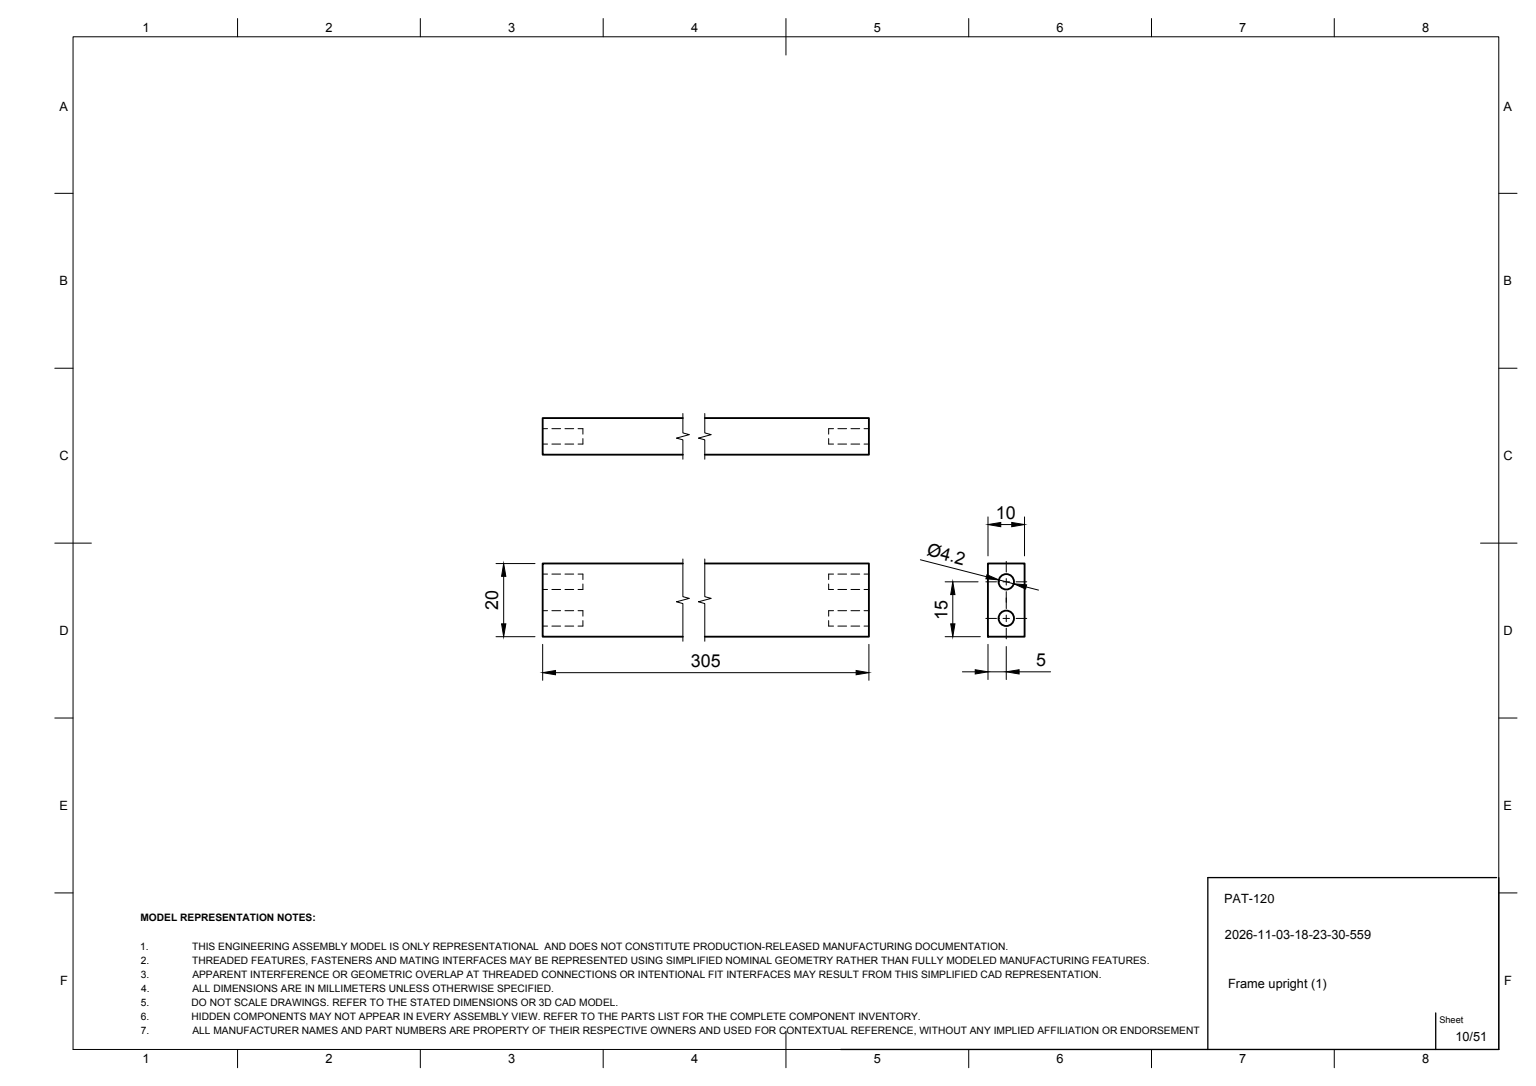
ISO-10303-21;
HEADER;
/* Generated by software containing ST-Developer
 * from STEP Tools, Inc. (www.steptools.com) 
 */

FILE_DESCRIPTION(
/* description */ ('Vibration shaker table dummy'),
/* implementation_level */ '2;1');

FILE_NAME(
/* name */ 'Frame upright (1).step',
/* time_stamp */ '2026-10-27T10:55:14-07:00',
/* author */ (''),
/* organization */ (''),
/* preprocessor_version */ 'ST-DEVELOPER v20.2',
/* originating_system */ 'Autodesk Translation Framework v15.17.0.0',
/* authorisation */ '');

FILE_SCHEMA (('AUTOMOTIVE_DESIGN { 1 0 10303 214 3 1 1 }'));
ENDSEC;

DATA;
#10=MECHANICAL_DESIGN_GEOMETRIC_PRESENTATION_REPRESENTATION('',(#691),#22394);
#599=SHAPE_REPRESENTATION_RELATIONSHIP('SRR','None',#22645,#645);
#645=ADVANCED_BREP_SHAPE_REPRESENTATION('',(#737),#22351);
#691=STYLED_ITEM('',(#22940),#737);
#737=MANIFOLD_SOLID_BREP('Body1',#9209);
#859=FACE_BOUND('',#2014,.T.);
#860=FACE_BOUND('',#2015,.T.);
#861=FACE_BOUND('',#2017,.T.);
#862=FACE_BOUND('',#2018,.T.);
#1094=PLANE('',#9937);
#1095=PLANE('',#9941);
#1096=PLANE('',#9945);
#1097=PLANE('',#9949);
#1098=PLANE('',#9950);
#1099=PLANE('',#9951);
#1100=PLANE('',#9952);
#1101=PLANE('',#9953);
#1102=PLANE('',#9954);
#1103=PLANE('',#9955);
#1419=FACE_OUTER_BOUND('',#2001,.T.);
#1420=FACE_OUTER_BOUND('',#2002,.T.);
#1421=FACE_OUTER_BOUND('',#2003,.T.);
#1422=FACE_OUTER_BOUND('',#2004,.T.);
#1423=FACE_OUTER_BOUND('',#2005,.T.);
#1424=FACE_OUTER_BOUND('',#2006,.T.);
#1425=FACE_OUTER_BOUND('',#2007,.T.);
#1426=FACE_OUTER_BOUND('',#2008,.T.);
#1427=FACE_OUTER_BOUND('',#2009,.T.);
#1428=FACE_OUTER_BOUND('',#2010,.T.);
#1429=FACE_OUTER_BOUND('',#2011,.T.);
#1430=FACE_OUTER_BOUND('',#2012,.T.);
#1431=FACE_OUTER_BOUND('',#2013,.T.);
#1432=FACE_OUTER_BOUND('',#2016,.T.);
#2001=EDGE_LOOP('',(#6630,#6631,#6632,#6633));
#2002=EDGE_LOOP('',(#6634));
#2003=EDGE_LOOP('',(#6635,#6636,#6637,#6638));
#2004=EDGE_LOOP('',(#6639));
#2005=EDGE_LOOP('',(#6640,#6641,#6642,#6643));
#2006=EDGE_LOOP('',(#6644));
#2007=EDGE_LOOP('',(#6645,#6646,#6647,#6648));
#2008=EDGE_LOOP('',(#6649));
#2009=EDGE_LOOP('',(#6650,#6651,#6652,#6653));
#2010=EDGE_LOOP('',(#6654,#6655,#6656,#6657));
#2011=EDGE_LOOP('',(#6658,#6659,#6660,#6661));
#2012=EDGE_LOOP('',(#6662,#6663,#6664,#6665));
#2013=EDGE_LOOP('',(#6666,#6667,#6668,#6669));
#2014=EDGE_LOOP('',(#6670));
#2015=EDGE_LOOP('',(#6671));
#2016=EDGE_LOOP('',(#6672,#6673,#6674,#6675));
#2017=EDGE_LOOP('',(#6676));
#2018=EDGE_LOOP('',(#6677));
#2726=LINE('',#14359,#3345);
#2727=LINE('',#14366,#3346);
#2728=LINE('',#14373,#3347);
#2729=LINE('',#14380,#3348);
#2730=LINE('',#14386,#3349);
#2731=LINE('',#14388,#3350);
#2732=LINE('',#14390,#3351);
#2733=LINE('',#14391,#3352);
#2734=LINE('',#14394,#3353);
#2735=LINE('',#14396,#3354);
#2736=LINE('',#14397,#3355);
#2737=LINE('',#14400,#3356);
#2738=LINE('',#14402,#3357);
#2739=LINE('',#14403,#3358);
#2740=LINE('',#14405,#3359);
#2741=LINE('',#14406,#3360);
#3345=VECTOR('',#11406,0.210000000000001);
#3346=VECTOR('',#11415,0.210000000000001);
#3347=VECTOR('',#11424,0.210000000000001);
#3348=VECTOR('',#11433,0.210000000000001);
#3349=VECTOR('',#11440,1.);
#3350=VECTOR('',#11441,1.);
#3351=VECTOR('',#11442,1.);
#3352=VECTOR('',#11443,1.);
#3353=VECTOR('',#11446,1.);
#3354=VECTOR('',#11447,1.);
#3355=VECTOR('',#11448,1.);
#3356=VECTOR('',#11451,1.);
#3357=VECTOR('',#11452,1.);
#3358=VECTOR('',#11453,1.);
#3359=VECTOR('',#11456,1.);
#3360=VECTOR('',#11457,1.);
#3948=CIRCLE('',#9935,0.210000000000001);
#3949=CIRCLE('',#9936,0.210000000000001);
#3950=CIRCLE('',#9939,0.210000000000001);
#3951=CIRCLE('',#9940,0.210000000000001);
#3952=CIRCLE('',#9943,0.210000000000001);
#3953=CIRCLE('',#9944,0.210000000000001);
#3954=CIRCLE('',#9947,0.210000000000001);
#3955=CIRCLE('',#9948,0.210000000000001);
#4495=VERTEX_POINT('',#14356);
#4496=VERTEX_POINT('',#14358);
#4497=VERTEX_POINT('',#14363);
#4498=VERTEX_POINT('',#14365);
#4499=VERTEX_POINT('',#14370);
#4500=VERTEX_POINT('',#14372);
#4501=VERTEX_POINT('',#14377);
#4502=VERTEX_POINT('',#14379);
#4503=VERTEX_POINT('',#14384);
#4504=VERTEX_POINT('',#14385);
#4505=VERTEX_POINT('',#14387);
#4506=VERTEX_POINT('',#14389);
#4507=VERTEX_POINT('',#14393);
#4508=VERTEX_POINT('',#14395);
#4509=VERTEX_POINT('',#14399);
#4510=VERTEX_POINT('',#14401);
#5308=EDGE_CURVE('',#4495,#4495,#3948,.T.);
#5309=EDGE_CURVE('',#4495,#4496,#2726,.T.);
#5310=EDGE_CURVE('',#4496,#4496,#3949,.T.);
#5311=EDGE_CURVE('',#4497,#4497,#3950,.T.);
#5312=EDGE_CURVE('',#4497,#4498,#2727,.T.);
#5313=EDGE_CURVE('',#4498,#4498,#3951,.T.);
#5314=EDGE_CURVE('',#4499,#4499,#3952,.T.);
#5315=EDGE_CURVE('',#4499,#4500,#2728,.T.);
#5316=EDGE_CURVE('',#4500,#4500,#3953,.T.);
#5317=EDGE_CURVE('',#4501,#4501,#3954,.T.);
#5318=EDGE_CURVE('',#4501,#4502,#2729,.T.);
#5319=EDGE_CURVE('',#4502,#4502,#3955,.T.);
#5320=EDGE_CURVE('',#4503,#4504,#2730,.T.);
#5321=EDGE_CURVE('',#4504,#4505,#2731,.T.);
#5322=EDGE_CURVE('',#4506,#4505,#2732,.T.);
#5323=EDGE_CURVE('',#4503,#4506,#2733,.T.);
#5324=EDGE_CURVE('',#4507,#4503,#2734,.T.);
#5325=EDGE_CURVE('',#4508,#4506,#2735,.T.);
#5326=EDGE_CURVE('',#4507,#4508,#2736,.T.);
#5327=EDGE_CURVE('',#4509,#4507,#2737,.T.);
#5328=EDGE_CURVE('',#4510,#4508,#2738,.T.);
#5329=EDGE_CURVE('',#4509,#4510,#2739,.T.);
#5330=EDGE_CURVE('',#4504,#4509,#2740,.T.);
#5331=EDGE_CURVE('',#4505,#4510,#2741,.T.);
#6630=ORIENTED_EDGE('',*,*,#5308,.F.);
#6631=ORIENTED_EDGE('',*,*,#5309,.T.);
#6632=ORIENTED_EDGE('',*,*,#5310,.F.);
#6633=ORIENTED_EDGE('',*,*,#5309,.F.);
#6634=ORIENTED_EDGE('',*,*,#5308,.T.);
#6635=ORIENTED_EDGE('',*,*,#5311,.F.);
#6636=ORIENTED_EDGE('',*,*,#5312,.T.);
#6637=ORIENTED_EDGE('',*,*,#5313,.F.);
#6638=ORIENTED_EDGE('',*,*,#5312,.F.);
#6639=ORIENTED_EDGE('',*,*,#5311,.T.);
#6640=ORIENTED_EDGE('',*,*,#5314,.F.);
#6641=ORIENTED_EDGE('',*,*,#5315,.T.);
#6642=ORIENTED_EDGE('',*,*,#5316,.T.);
#6643=ORIENTED_EDGE('',*,*,#5315,.F.);
#6644=ORIENTED_EDGE('',*,*,#5316,.F.);
#6645=ORIENTED_EDGE('',*,*,#5317,.F.);
#6646=ORIENTED_EDGE('',*,*,#5318,.T.);
#6647=ORIENTED_EDGE('',*,*,#5319,.T.);
#6648=ORIENTED_EDGE('',*,*,#5318,.F.);
#6649=ORIENTED_EDGE('',*,*,#5319,.F.);
#6650=ORIENTED_EDGE('',*,*,#5320,.T.);
#6651=ORIENTED_EDGE('',*,*,#5321,.T.);
#6652=ORIENTED_EDGE('',*,*,#5322,.F.);
#6653=ORIENTED_EDGE('',*,*,#5323,.F.);
#6654=ORIENTED_EDGE('',*,*,#5324,.T.);
#6655=ORIENTED_EDGE('',*,*,#5323,.T.);
#6656=ORIENTED_EDGE('',*,*,#5325,.F.);
#6657=ORIENTED_EDGE('',*,*,#5326,.F.);
#6658=ORIENTED_EDGE('',*,*,#5327,.T.);
#6659=ORIENTED_EDGE('',*,*,#5326,.T.);
#6660=ORIENTED_EDGE('',*,*,#5328,.F.);
#6661=ORIENTED_EDGE('',*,*,#5329,.F.);
#6662=ORIENTED_EDGE('',*,*,#5330,.T.);
#6663=ORIENTED_EDGE('',*,*,#5329,.T.);
#6664=ORIENTED_EDGE('',*,*,#5331,.F.);
#6665=ORIENTED_EDGE('',*,*,#5321,.F.);
#6666=ORIENTED_EDGE('',*,*,#5331,.T.);
#6667=ORIENTED_EDGE('',*,*,#5328,.T.);
#6668=ORIENTED_EDGE('',*,*,#5325,.T.);
#6669=ORIENTED_EDGE('',*,*,#5322,.T.);
#6670=ORIENTED_EDGE('',*,*,#5310,.T.);
#6671=ORIENTED_EDGE('',*,*,#5313,.T.);
#6672=ORIENTED_EDGE('',*,*,#5330,.F.);
#6673=ORIENTED_EDGE('',*,*,#5320,.F.);
#6674=ORIENTED_EDGE('',*,*,#5324,.F.);
#6675=ORIENTED_EDGE('',*,*,#5327,.F.);
#6676=ORIENTED_EDGE('',*,*,#5314,.T.);
#6677=ORIENTED_EDGE('',*,*,#5317,.T.);
#8550=CYLINDRICAL_SURFACE('',#9934,0.210000000000001);
#8551=CYLINDRICAL_SURFACE('',#9938,0.210000000000001);
#8552=CYLINDRICAL_SURFACE('',#9942,0.210000000000001);
#8553=CYLINDRICAL_SURFACE('',#9946,0.210000000000001);
#8784=ADVANCED_FACE('',(#1419),#8550,.F.);
#8785=ADVANCED_FACE('',(#1420),#1094,.T.);
#8786=ADVANCED_FACE('',(#1421),#8551,.F.);
#8787=ADVANCED_FACE('',(#1422),#1095,.T.);
#8788=ADVANCED_FACE('',(#1423),#8552,.F.);
#8789=ADVANCED_FACE('',(#1424),#1096,.F.);
#8790=ADVANCED_FACE('',(#1425),#8553,.F.);
#8791=ADVANCED_FACE('',(#1426),#1097,.F.);
#8792=ADVANCED_FACE('',(#1427),#1098,.T.);
#8793=ADVANCED_FACE('',(#1428),#1099,.T.);
#8794=ADVANCED_FACE('',(#1429),#1100,.T.);
#8795=ADVANCED_FACE('',(#1430),#1101,.T.);
#8796=ADVANCED_FACE('',(#1431,#859,#860),#1102,.T.);
#8797=ADVANCED_FACE('',(#1432,#861,#862),#1103,.F.);
#9209=CLOSED_SHELL('',(#8784,#8785,#8786,#8787,#8788,#8789,#8790,#8791,
#8792,#8793,#8794,#8795,#8796,#8797));
#9933=AXIS2_PLACEMENT_3D('',#14354,#11400,#11401);
#9934=AXIS2_PLACEMENT_3D('',#14355,#11402,#11403);
#9935=AXIS2_PLACEMENT_3D('',#14357,#11404,#11405);
#9936=AXIS2_PLACEMENT_3D('',#14360,#11407,#11408);
#9937=AXIS2_PLACEMENT_3D('',#14361,#11409,#11410);
#9938=AXIS2_PLACEMENT_3D('',#14362,#11411,#11412);
#9939=AXIS2_PLACEMENT_3D('',#14364,#11413,#11414);
#9940=AXIS2_PLACEMENT_3D('',#14367,#11416,#11417);
#9941=AXIS2_PLACEMENT_3D('',#14368,#11418,#11419);
#9942=AXIS2_PLACEMENT_3D('',#14369,#11420,#11421);
#9943=AXIS2_PLACEMENT_3D('',#14371,#11422,#11423);
#9944=AXIS2_PLACEMENT_3D('',#14374,#11425,#11426);
#9945=AXIS2_PLACEMENT_3D('',#14375,#11427,#11428);
#9946=AXIS2_PLACEMENT_3D('',#14376,#11429,#11430);
#9947=AXIS2_PLACEMENT_3D('',#14378,#11431,#11432);
#9948=AXIS2_PLACEMENT_3D('',#14381,#11434,#11435);
#9949=AXIS2_PLACEMENT_3D('',#14382,#11436,#11437);
#9950=AXIS2_PLACEMENT_3D('',#14383,#11438,#11439);
#9951=AXIS2_PLACEMENT_3D('',#14392,#11444,#11445);
#9952=AXIS2_PLACEMENT_3D('',#14398,#11449,#11450);
#9953=AXIS2_PLACEMENT_3D('',#14404,#11454,#11455);
#9954=AXIS2_PLACEMENT_3D('',#14407,#11458,#11459);
#9955=AXIS2_PLACEMENT_3D('',#14408,#11460,#11461);
#11400=DIRECTION('axis',(0.,0.,1.));
#11401=DIRECTION('refdir',(1.,0.,0.));
#11402=DIRECTION('center_axis',(0.,0.,1.));
#11403=DIRECTION('ref_axis',(1.,0.,0.));
#11404=DIRECTION('center_axis',(0.,0.,1.));
#11405=DIRECTION('ref_axis',(1.,0.,0.));
#11406=DIRECTION('',(0.,0.,1.));
#11407=DIRECTION('center_axis',(0.,0.,-1.));
#11408=DIRECTION('ref_axis',(1.,0.,0.));
#11409=DIRECTION('center_axis',(0.,0.,1.));
#11410=DIRECTION('ref_axis',(1.,0.,0.));
#11411=DIRECTION('center_axis',(0.,0.,1.));
#11412=DIRECTION('ref_axis',(1.,0.,0.));
#11413=DIRECTION('center_axis',(0.,0.,1.));
#11414=DIRECTION('ref_axis',(1.,0.,0.));
#11415=DIRECTION('',(0.,0.,1.));
#11416=DIRECTION('center_axis',(0.,0.,-1.));
#11417=DIRECTION('ref_axis',(1.,0.,0.));
#11418=DIRECTION('center_axis',(0.,0.,1.));
#11419=DIRECTION('ref_axis',(1.,0.,0.));
#11420=DIRECTION('center_axis',(0.,0.,1.));
#11421=DIRECTION('ref_axis',(1.,0.,0.));
#11422=DIRECTION('center_axis',(0.,0.,1.));
#11423=DIRECTION('ref_axis',(1.,0.,0.));
#11424=DIRECTION('',(0.,0.,1.));
#11425=DIRECTION('center_axis',(0.,0.,1.));
#11426=DIRECTION('ref_axis',(1.,0.,0.));
#11427=DIRECTION('center_axis',(0.,0.,1.));
#11428=DIRECTION('ref_axis',(1.,0.,0.));
#11429=DIRECTION('center_axis',(0.,0.,1.));
#11430=DIRECTION('ref_axis',(1.,0.,0.));
#11431=DIRECTION('center_axis',(0.,0.,1.));
#11432=DIRECTION('ref_axis',(1.,0.,0.));
#11433=DIRECTION('',(0.,0.,1.));
#11434=DIRECTION('center_axis',(0.,0.,1.));
#11435=DIRECTION('ref_axis',(1.,0.,0.));
#11436=DIRECTION('center_axis',(0.,0.,1.));
#11437=DIRECTION('ref_axis',(1.,0.,0.));
#11438=DIRECTION('center_axis',(0.,1.,0.));
#11439=DIRECTION('ref_axis',(-1.,0.,0.));
#11440=DIRECTION('',(-1.,0.,0.));
#11441=DIRECTION('',(0.,0.,1.));
#11442=DIRECTION('',(-1.,0.,0.));
#11443=DIRECTION('',(0.,0.,1.));
#11444=DIRECTION('center_axis',(1.,0.,0.));
#11445=DIRECTION('ref_axis',(0.,1.,0.));
#11446=DIRECTION('',(0.,1.,0.));
#11447=DIRECTION('',(0.,1.,0.));
#11448=DIRECTION('',(0.,0.,1.));
#11449=DIRECTION('center_axis',(0.,-1.,0.));
#11450=DIRECTION('ref_axis',(1.,0.,0.));
#11451=DIRECTION('',(1.,0.,0.));
#11452=DIRECTION('',(1.,0.,0.));
#11453=DIRECTION('',(0.,0.,1.));
#11454=DIRECTION('center_axis',(-1.,0.,0.));
#11455=DIRECTION('ref_axis',(0.,-1.,0.));
#11456=DIRECTION('',(0.,-1.,0.));
#11457=DIRECTION('',(0.,-1.,0.));
#11458=DIRECTION('center_axis',(0.,0.,1.));
#11459=DIRECTION('ref_axis',(1.,0.,0.));
#11460=DIRECTION('center_axis',(0.,0.,1.));
#11461=DIRECTION('ref_axis',(1.,0.,0.));
#14354=CARTESIAN_POINT('',(0.,0.,0.));
#14355=CARTESIAN_POINT('Origin',(9.5,10.,29.4));
#14356=CARTESIAN_POINT('',(9.29,10.,29.4));
#14357=CARTESIAN_POINT('Origin',(9.5,10.,29.4));
#14358=CARTESIAN_POINT('',(9.29,10.,30.5));
#14359=CARTESIAN_POINT('',(9.29,10.,29.4));
#14360=CARTESIAN_POINT('Origin',(9.5,10.,30.5));
#14361=CARTESIAN_POINT('Origin',(9.5,10.,29.4));
#14362=CARTESIAN_POINT('Origin',(9.5,11.,29.4));
#14363=CARTESIAN_POINT('',(9.29,11.,29.4));
#14364=CARTESIAN_POINT('Origin',(9.5,11.,29.4));
#14365=CARTESIAN_POINT('',(9.29,11.,30.5));
#14366=CARTESIAN_POINT('',(9.29,11.,29.4));
#14367=CARTESIAN_POINT('Origin',(9.5,11.,30.5));
#14368=CARTESIAN_POINT('Origin',(9.5,11.,29.4));
#14369=CARTESIAN_POINT('Origin',(9.5,10.,-0.1));
#14370=CARTESIAN_POINT('',(9.29,10.,0.));
#14371=CARTESIAN_POINT('Origin',(9.5,10.,0.));
#14372=CARTESIAN_POINT('',(9.29,10.,1.1));
#14373=CARTESIAN_POINT('',(9.29,10.,-0.1));
#14374=CARTESIAN_POINT('Origin',(9.5,10.,1.1));
#14375=CARTESIAN_POINT('Origin',(9.5,10.,1.1));
#14376=CARTESIAN_POINT('Origin',(9.5,11.,-0.1));
#14377=CARTESIAN_POINT('',(9.29,11.,0.));
#14378=CARTESIAN_POINT('Origin',(9.5,11.,0.));
#14379=CARTESIAN_POINT('',(9.29,11.,1.1));
#14380=CARTESIAN_POINT('',(9.29,11.,-0.1));
#14381=CARTESIAN_POINT('Origin',(9.5,11.,1.1));
#14382=CARTESIAN_POINT('Origin',(9.5,11.,1.1));
#14383=CARTESIAN_POINT('Origin',(10.,11.5,0.));
#14384=CARTESIAN_POINT('',(10.,11.5,0.));
#14385=CARTESIAN_POINT('',(9.,11.5,0.));
#14386=CARTESIAN_POINT('',(10.,11.5,0.));
#14387=CARTESIAN_POINT('',(9.,11.5,30.5));
#14388=CARTESIAN_POINT('',(9.,11.5,0.));
#14389=CARTESIAN_POINT('',(10.,11.5,30.5));
#14390=CARTESIAN_POINT('',(10.,11.5,30.5));
#14391=CARTESIAN_POINT('',(10.,11.5,0.));
#14392=CARTESIAN_POINT('Origin',(10.,9.5,0.));
#14393=CARTESIAN_POINT('',(10.,9.5,0.));
#14394=CARTESIAN_POINT('',(10.,9.5,0.));
#14395=CARTESIAN_POINT('',(10.,9.5,30.5));
#14396=CARTESIAN_POINT('',(10.,9.5,30.5));
#14397=CARTESIAN_POINT('',(10.,9.5,0.));
#14398=CARTESIAN_POINT('Origin',(9.,9.5,0.));
#14399=CARTESIAN_POINT('',(9.,9.5,0.));
#14400=CARTESIAN_POINT('',(9.,9.5,0.));
#14401=CARTESIAN_POINT('',(9.,9.5,30.5));
#14402=CARTESIAN_POINT('',(9.,9.5,30.5));
#14403=CARTESIAN_POINT('',(9.,9.5,0.));
#14404=CARTESIAN_POINT('Origin',(9.,11.5,0.));
#14405=CARTESIAN_POINT('',(9.,11.5,0.));
#14406=CARTESIAN_POINT('',(9.,11.5,30.5));
#14407=CARTESIAN_POINT('Origin',(9.5,10.5,30.5));
#14408=CARTESIAN_POINT('Origin',(9.5,10.5,0.));
#22300=UNCERTAINTY_MEASURE_WITH_UNIT(LENGTH_MEASURE(0.001),#22395,
'DISTANCE_ACCURACY_VALUE',
'Maximum model space distance between geometric entities at asserted c
onnectivities');
#22343=UNCERTAINTY_MEASURE_WITH_UNIT(LENGTH_MEASURE(0.001),#22395,
'DISTANCE_ACCURACY_VALUE',
'Maximum model space distance between geometric entities at asserted c
onnectivities');
#22351=(
GEOMETRIC_REPRESENTATION_CONTEXT(3)
GLOBAL_UNCERTAINTY_ASSIGNED_CONTEXT((#22300))
GLOBAL_UNIT_ASSIGNED_CONTEXT((#22395,#22397,#22398))
REPRESENTATION_CONTEXT('','3D')
);
#22394=(
GEOMETRIC_REPRESENTATION_CONTEXT(3)
GLOBAL_UNCERTAINTY_ASSIGNED_CONTEXT((#22343))
GLOBAL_UNIT_ASSIGNED_CONTEXT((#22395,#22397,#22398))
REPRESENTATION_CONTEXT('','3D')
);
#22395=(
LENGTH_UNIT()
NAMED_UNIT(*)
SI_UNIT(.CENTI.,.METRE.)
);
#22397=(
NAMED_UNIT(*)
PLANE_ANGLE_UNIT()
SI_UNIT($,.RADIAN.)
);
#22398=(
NAMED_UNIT(*)
SI_UNIT($,.STERADIAN.)
SOLID_ANGLE_UNIT()
);
#22406=SHAPE_DEFINITION_REPRESENTATION(#22456,#22645);
#22456=PRODUCT_DEFINITION_SHAPE('',$,#22696);
#22645=SHAPE_REPRESENTATION('',(#9933),#22351);
#22688=PRODUCT_DEFINITION_CONTEXT('part definition',#22840,'design');
#22696=PRODUCT_DEFINITION('Frame upright (1)','Frame upright (1)',#22746,
#22688);
#22746=PRODUCT_DEFINITION_FORMATION('',$,#22849);
#22840=APPLICATION_CONTEXT(
'Core Data for Automotive Mechanical Design Process');
#22841=PRODUCT_CONTEXT('part definition',#22840,'mechanical');
#22849=PRODUCT('Frame upright (1)','Frame upright (1)','Frame upright (1)',(#22841));
#22934=COLOUR_RGB('Dark Blue',0.08,0.2,0.34);
#22935=FILL_AREA_STYLE_COLOUR('',#22934);
#22936=FILL_AREA_STYLE('',(#22935));
#22937=SURFACE_STYLE_FILL_AREA(#22936);
#22938=SURFACE_SIDE_STYLE('',(#22937));
#22939=SURFACE_STYLE_USAGE(.BOTH.,#22938);
#22940=PRESENTATION_STYLE_ASSIGNMENT((#22939));
ENDSEC;
END-ISO-10303-21;
